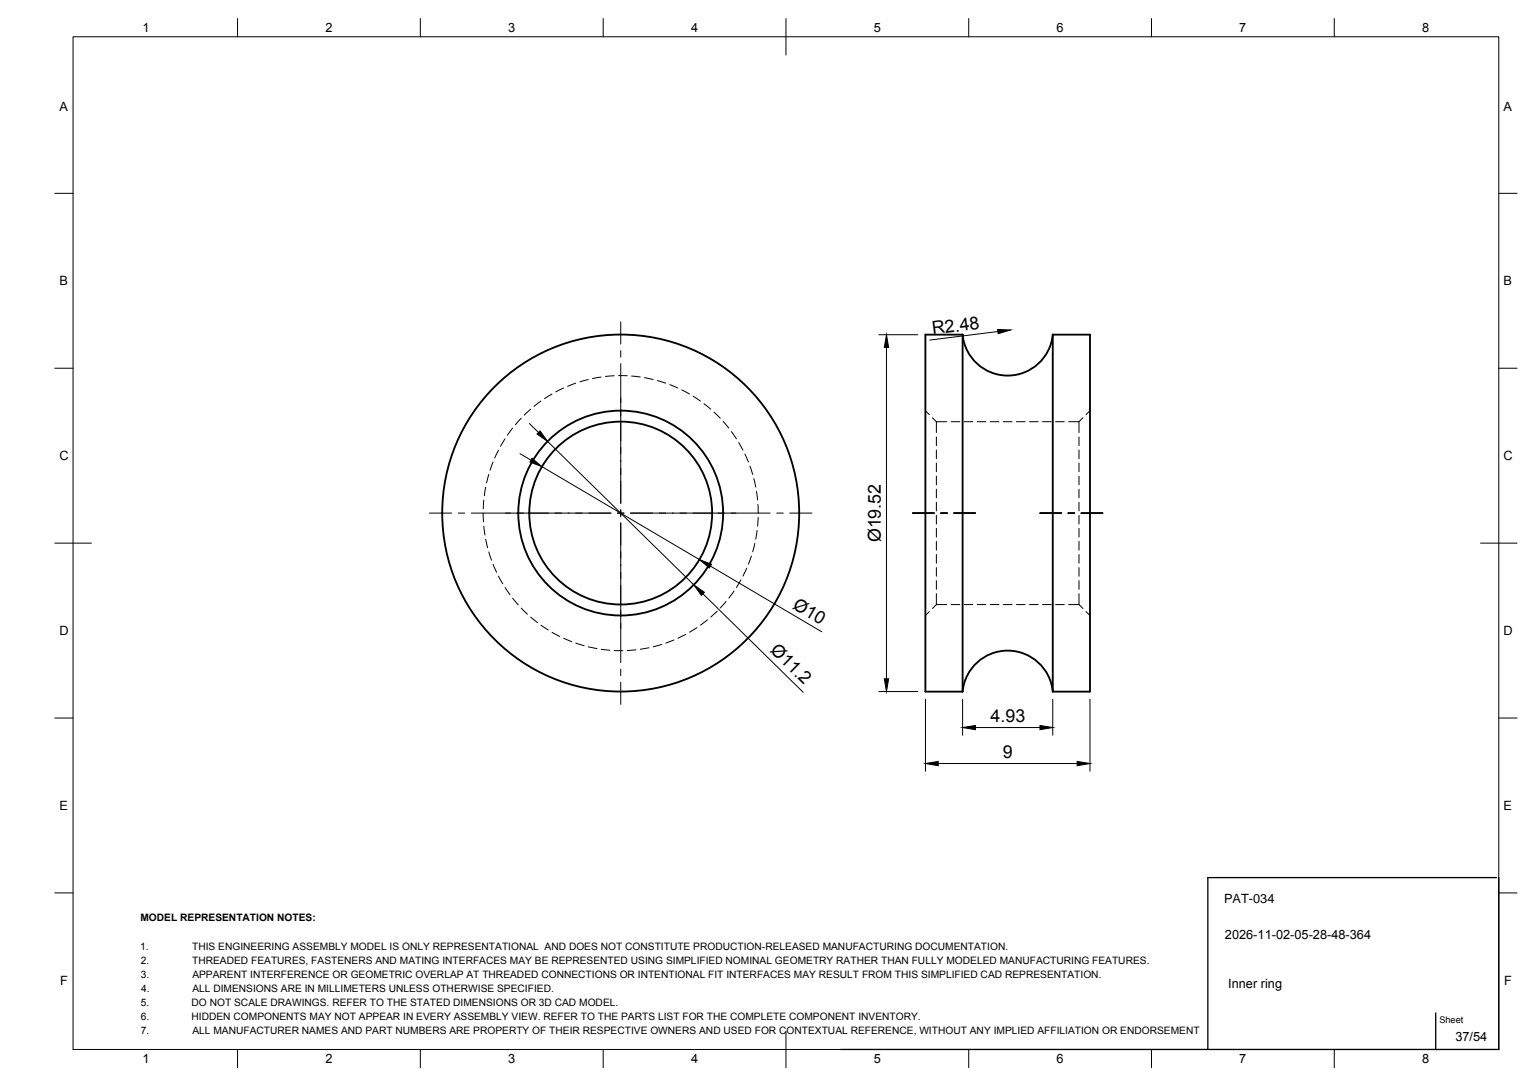
ISO-10303-21;
HEADER;
/* Generated by software containing ST-Developer
 * from STEP Tools, Inc. (www.steptools.com) 
 */

FILE_DESCRIPTION(
/* description */ ('Fatigue rig crank-slider'),
/* implementation_level */ '2;1');

FILE_NAME(
/* name */ 'Inner ring.step',
/* time_stamp */ '2026-10-28T03:24:50-07:00',
/* author */ (''),
/* organization */ (''),
/* preprocessor_version */ 'ST-DEVELOPER v20.2',
/* originating_system */ 'Autodesk Translation Framework v15.17.0.0',
/* authorisation */ '');

FILE_SCHEMA (('AUTOMOTIVE_DESIGN { 1 0 10303 214 3 1 1 }'));
ENDSEC;

DATA;
#10=MECHANICAL_DESIGN_GEOMETRIC_PRESENTATION_REPRESENTATION('',(#620),#16911);
#11=TOROIDAL_SURFACE('',#10108,1.,0.247676);
#22=CONICAL_SURFACE('',#10119,0.53,0.785398163397448);
#23=CONICAL_SURFACE('',#10126,0.53,0.785398163397448);
#519=SHAPE_REPRESENTATION_RELATIONSHIP('SRR','None',#17162,#569);
#569=ADVANCED_BREP_SHAPE_REPRESENTATION('',(#677),#16891);
#620=STYLED_ITEM('',(#17487),#677);
#677=MANIFOLD_SOLID_BREP('Body1',#8913);
#854=FACE_BOUND('',#2224,.T.);
#855=FACE_BOUND('',#2227,.T.);
#1094=PLANE('',#10121);
#1095=PLANE('',#10124);
#1542=FACE_OUTER_BOUND('',#2219,.T.);
#1543=FACE_OUTER_BOUND('',#2220,.T.);
#1544=FACE_OUTER_BOUND('',#2221,.T.);
#1545=FACE_OUTER_BOUND('',#2222,.T.);
#1546=FACE_OUTER_BOUND('',#2223,.T.);
#1547=FACE_OUTER_BOUND('',#2225,.T.);
#1548=FACE_OUTER_BOUND('',#2226,.T.);
#1549=FACE_OUTER_BOUND('',#2228,.T.);
#2219=EDGE_LOOP('',(#7340,#7341,#7342,#7343,#7344,#7345));
#2220=EDGE_LOOP('',(#7346,#7347,#7348,#7349,#7350));
#2221=EDGE_LOOP('',(#7351,#7352,#7353,#7354));
#2222=EDGE_LOOP('',(#7355,#7356,#7357,#7358));
#2223=EDGE_LOOP('',(#7359));
#2224=EDGE_LOOP('',(#7360));
#2225=EDGE_LOOP('',(#7361,#7362,#7363,#7364,#7365));
#2226=EDGE_LOOP('',(#7366));
#2227=EDGE_LOOP('',(#7367));
#2228=EDGE_LOOP('',(#7368,#7369,#7370,#7371));
#2847=LINE('',#15442,#3493);
#2848=LINE('',#15448,#3494);
#2849=LINE('',#15452,#3495);
#2850=LINE('',#15458,#3496);
#2851=LINE('',#15463,#3497);
#3493=VECTOR('',#12197,0.976185);
#3494=VECTOR('',#12204,0.5);
#3495=VECTOR('',#12209,0.53);
#3496=VECTOR('',#12218,0.976185);
#3497=VECTOR('',#12225,0.53);
#4001=CIRCLE('',#10109,0.976185);
#4002=CIRCLE('',#10110,0.976185);
#4003=CIRCLE('',#10111,0.247676);
#4004=CIRCLE('',#10112,0.976185);
#4005=CIRCLE('',#10113,0.976185);
#4006=CIRCLE('',#10115,0.976185);
#4007=CIRCLE('',#10117,0.5);
#4008=CIRCLE('',#10118,0.5);
#4009=CIRCLE('',#10120,0.56);
#4010=CIRCLE('',#10123,0.976185);
#4011=CIRCLE('',#10125,0.56);
#4605=VERTEX_POINT('',#15431);
#4606=VERTEX_POINT('',#15432);
#4607=VERTEX_POINT('',#15435);
#4608=VERTEX_POINT('',#15437);
#4609=VERTEX_POINT('',#15441);
#4610=VERTEX_POINT('',#15445);
#4611=VERTEX_POINT('',#15447);
#4612=VERTEX_POINT('',#15451);
#4613=VERTEX_POINT('',#15456);
#4614=VERTEX_POINT('',#15460);
#5568=EDGE_CURVE('',#4605,#4606,#4001,.T.);
#5569=EDGE_CURVE('',#4606,#4605,#4002,.T.);
#5570=EDGE_CURVE('',#4606,#4607,#4003,.T.);
#5571=EDGE_CURVE('',#4608,#4607,#4004,.T.);
#5572=EDGE_CURVE('',#4607,#4608,#4005,.T.);
#5573=EDGE_CURVE('',#4608,#4609,#2847,.T.);
#5574=EDGE_CURVE('',#4609,#4609,#4006,.T.);
#5575=EDGE_CURVE('',#4610,#4610,#4007,.T.);
#5576=EDGE_CURVE('',#4610,#4611,#2848,.T.);
#5577=EDGE_CURVE('',#4611,#4611,#4008,.T.);
#5578=EDGE_CURVE('',#4611,#4612,#2849,.T.);
#5579=EDGE_CURVE('',#4612,#4612,#4009,.T.);
#5580=EDGE_CURVE('',#4613,#4613,#4010,.T.);
#5581=EDGE_CURVE('',#4613,#4605,#2850,.T.);
#5582=EDGE_CURVE('',#4614,#4614,#4011,.T.);
#5583=EDGE_CURVE('',#4614,#4610,#2851,.T.);
#7340=ORIENTED_EDGE('',*,*,#5568,.F.);
#7341=ORIENTED_EDGE('',*,*,#5569,.F.);
#7342=ORIENTED_EDGE('',*,*,#5570,.T.);
#7343=ORIENTED_EDGE('',*,*,#5571,.F.);
#7344=ORIENTED_EDGE('',*,*,#5572,.F.);
#7345=ORIENTED_EDGE('',*,*,#5570,.F.);
#7346=ORIENTED_EDGE('',*,*,#5571,.T.);
#7347=ORIENTED_EDGE('',*,*,#5572,.T.);
#7348=ORIENTED_EDGE('',*,*,#5573,.T.);
#7349=ORIENTED_EDGE('',*,*,#5574,.T.);
#7350=ORIENTED_EDGE('',*,*,#5573,.F.);
#7351=ORIENTED_EDGE('',*,*,#5575,.T.);
#7352=ORIENTED_EDGE('',*,*,#5576,.T.);
#7353=ORIENTED_EDGE('',*,*,#5577,.F.);
#7354=ORIENTED_EDGE('',*,*,#5576,.F.);
#7355=ORIENTED_EDGE('',*,*,#5577,.T.);
#7356=ORIENTED_EDGE('',*,*,#5578,.T.);
#7357=ORIENTED_EDGE('',*,*,#5579,.F.);
#7358=ORIENTED_EDGE('',*,*,#5578,.F.);
#7359=ORIENTED_EDGE('',*,*,#5574,.F.);
#7360=ORIENTED_EDGE('',*,*,#5579,.T.);
#7361=ORIENTED_EDGE('',*,*,#5580,.F.);
#7362=ORIENTED_EDGE('',*,*,#5581,.T.);
#7363=ORIENTED_EDGE('',*,*,#5568,.T.);
#7364=ORIENTED_EDGE('',*,*,#5569,.T.);
#7365=ORIENTED_EDGE('',*,*,#5581,.F.);
#7366=ORIENTED_EDGE('',*,*,#5580,.T.);
#7367=ORIENTED_EDGE('',*,*,#5582,.F.);
#7368=ORIENTED_EDGE('',*,*,#5582,.T.);
#7369=ORIENTED_EDGE('',*,*,#5583,.T.);
#7370=ORIENTED_EDGE('',*,*,#5575,.F.);
#7371=ORIENTED_EDGE('',*,*,#5583,.F.);
#8313=CYLINDRICAL_SURFACE('',#10114,0.976185);
#8314=CYLINDRICAL_SURFACE('',#10116,0.5);
#8315=CYLINDRICAL_SURFACE('',#10122,0.976185);
#8680=ADVANCED_FACE('',(#1542),#11,.F.);
#8681=ADVANCED_FACE('',(#1543),#8313,.T.);
#8682=ADVANCED_FACE('',(#1544),#8314,.F.);
#8683=ADVANCED_FACE('',(#1545),#22,.F.);
#8684=ADVANCED_FACE('',(#1546,#854),#1094,.T.);
#8685=ADVANCED_FACE('',(#1547),#8315,.T.);
#8686=ADVANCED_FACE('',(#1548,#855),#1095,.T.);
#8687=ADVANCED_FACE('',(#1549),#23,.F.);
#8913=CLOSED_SHELL('',(#8680,#8681,#8682,#8683,#8684,#8685,#8686,#8687));
#10107=AXIS2_PLACEMENT_3D('',#15429,#12181,#12182);
#10108=AXIS2_PLACEMENT_3D('',#15430,#12183,#12184);
#10109=AXIS2_PLACEMENT_3D('',#15433,#12185,#12186);
#10110=AXIS2_PLACEMENT_3D('',#15434,#12187,#12188);
#10111=AXIS2_PLACEMENT_3D('',#15436,#12189,#12190);
#10112=AXIS2_PLACEMENT_3D('',#15438,#12191,#12192);
#10113=AXIS2_PLACEMENT_3D('',#15439,#12193,#12194);
#10114=AXIS2_PLACEMENT_3D('',#15440,#12195,#12196);
#10115=AXIS2_PLACEMENT_3D('',#15443,#12198,#12199);
#10116=AXIS2_PLACEMENT_3D('',#15444,#12200,#12201);
#10117=AXIS2_PLACEMENT_3D('',#15446,#12202,#12203);
#10118=AXIS2_PLACEMENT_3D('',#15449,#12205,#12206);
#10119=AXIS2_PLACEMENT_3D('',#15450,#12207,#12208);
#10120=AXIS2_PLACEMENT_3D('',#15453,#12210,#12211);
#10121=AXIS2_PLACEMENT_3D('',#15454,#12212,#12213);
#10122=AXIS2_PLACEMENT_3D('',#15455,#12214,#12215);
#10123=AXIS2_PLACEMENT_3D('',#15457,#12216,#12217);
#10124=AXIS2_PLACEMENT_3D('',#15459,#12219,#12220);
#10125=AXIS2_PLACEMENT_3D('',#15461,#12221,#12222);
#10126=AXIS2_PLACEMENT_3D('',#15462,#12223,#12224);
#12181=DIRECTION('axis',(0.,0.,1.));
#12182=DIRECTION('refdir',(1.,0.,0.));
#12183=DIRECTION('center_axis',(0.,-1.,0.));
#12184=DIRECTION('ref_axis',(0.,0.,-1.));
#12185=DIRECTION('center_axis',(0.,-1.,0.));
#12186=DIRECTION('ref_axis',(1.,0.,0.));
#12187=DIRECTION('center_axis',(0.,-1.,0.));
#12188=DIRECTION('ref_axis',(1.,0.,0.));
#12189=DIRECTION('center_axis',(1.,0.,1.22464679914735E-16));
#12190=DIRECTION('ref_axis',(-1.22464679914735E-16,0.,1.));
#12191=DIRECTION('center_axis',(0.,1.,0.));
#12192=DIRECTION('ref_axis',(1.,0.,0.));
#12193=DIRECTION('center_axis',(0.,1.,0.));
#12194=DIRECTION('ref_axis',(1.,0.,0.));
#12195=DIRECTION('center_axis',(0.,-1.,0.));
#12196=DIRECTION('ref_axis',(1.,0.,0.));
#12197=DIRECTION('',(0.,1.,0.));
#12198=DIRECTION('center_axis',(0.,-1.,0.));
#12199=DIRECTION('ref_axis',(1.,0.,0.));
#12200=DIRECTION('center_axis',(0.,-1.,0.));
#12201=DIRECTION('ref_axis',(1.,0.,0.));
#12202=DIRECTION('center_axis',(0.,-1.,0.));
#12203=DIRECTION('ref_axis',(1.,0.,0.));
#12204=DIRECTION('',(0.,1.,0.));
#12205=DIRECTION('center_axis',(0.,-1.,0.));
#12206=DIRECTION('ref_axis',(1.,0.,0.));
#12207=DIRECTION('center_axis',(0.,1.,0.));
#12208=DIRECTION('ref_axis',(1.,0.,0.));
#12209=DIRECTION('',(-0.707106781186547,0.707106781186548,-8.65956056235493E-17));
#12210=DIRECTION('center_axis',(0.,-1.,0.));
#12211=DIRECTION('ref_axis',(1.,0.,0.));
#12212=DIRECTION('center_axis',(0.,1.,0.));
#12213=DIRECTION('ref_axis',(0.,0.,1.));
#12214=DIRECTION('center_axis',(0.,-1.,0.));
#12215=DIRECTION('ref_axis',(1.,0.,0.));
#12216=DIRECTION('center_axis',(0.,-1.,0.));
#12217=DIRECTION('ref_axis',(1.,0.,0.));
#12218=DIRECTION('',(0.,1.,0.));
#12219=DIRECTION('center_axis',(0.,-1.,0.));
#12220=DIRECTION('ref_axis',(0.,0.,-1.));
#12221=DIRECTION('center_axis',(0.,-1.,0.));
#12222=DIRECTION('ref_axis',(1.,0.,0.));
#12223=DIRECTION('center_axis',(0.,-1.,0.));
#12224=DIRECTION('ref_axis',(1.,0.,0.));
#12225=DIRECTION('',(0.707106781186547,0.707106781186548,8.65956056235493E-17));
#15429=CARTESIAN_POINT('',(0.,0.,0.));
#15430=CARTESIAN_POINT('Origin',(0.,0.,0.));
#15431=CARTESIAN_POINT('',(-0.976185,-0.246528389340863,-1.19548183562566E-16));
#15432=CARTESIAN_POINT('',(-1.19548183562566E-16,-0.246528389340863,0.976185));
#15433=CARTESIAN_POINT('Origin',(0.,-0.246528389340863,0.));
#15434=CARTESIAN_POINT('Origin',(0.,-0.246528389340863,0.));
#15435=CARTESIAN_POINT('',(-1.19548183562566E-16,0.246528389340863,0.976185));
#15436=CARTESIAN_POINT('Origin',(-1.22464679914735E-16,0.,1.));
#15437=CARTESIAN_POINT('',(-0.976185,0.246528389340863,1.19548183562566E-16));
#15438=CARTESIAN_POINT('Origin',(0.,0.246528389340863,0.));
#15439=CARTESIAN_POINT('Origin',(0.,0.246528389340863,0.));
#15440=CARTESIAN_POINT('Origin',(0.,0.,0.));
#15441=CARTESIAN_POINT('',(-0.976185,0.45,-1.19548183562566E-16));
#15442=CARTESIAN_POINT('',(-0.976185,0.,-1.19548183562566E-16));
#15443=CARTESIAN_POINT('Origin',(0.,0.45,0.));
#15444=CARTESIAN_POINT('Origin',(0.,0.,0.));
#15445=CARTESIAN_POINT('',(-0.5,-0.39,-6.12323399573677E-17));
#15446=CARTESIAN_POINT('Origin',(0.,-0.39,0.));
#15447=CARTESIAN_POINT('',(-0.5,0.39,-6.12323399573677E-17));
#15448=CARTESIAN_POINT('',(-0.5,0.,-6.12323399573677E-17));
#15449=CARTESIAN_POINT('Origin',(0.,0.39,0.));
#15450=CARTESIAN_POINT('Origin',(0.,0.42,0.));
#15451=CARTESIAN_POINT('',(-0.56,0.45,-6.85802207522518E-17));
#15452=CARTESIAN_POINT('',(-0.53,0.42,-6.49062803548097E-17));
#15453=CARTESIAN_POINT('Origin',(0.,0.45,0.));
#15454=CARTESIAN_POINT('Origin',(0.976185,0.45,0.));
#15455=CARTESIAN_POINT('Origin',(0.,0.,0.));
#15456=CARTESIAN_POINT('',(-0.976185,-0.45,-1.19548183562566E-16));
#15457=CARTESIAN_POINT('Origin',(0.,-0.45,0.));
#15458=CARTESIAN_POINT('',(-0.976185,0.,-1.19548183562566E-16));
#15459=CARTESIAN_POINT('Origin',(0.56,-0.45,0.));
#15460=CARTESIAN_POINT('',(-0.56,-0.45,-6.85802207522518E-17));
#15461=CARTESIAN_POINT('Origin',(0.,-0.45,0.));
#15462=CARTESIAN_POINT('Origin',(0.,-0.42,0.));
#15463=CARTESIAN_POINT('',(-0.53,-0.42,-6.49062803548097E-17));
#16832=UNCERTAINTY_MEASURE_WITH_UNIT(LENGTH_MEASURE(0.001),#16912,
'DISTANCE_ACCURACY_VALUE',
'Maximum model space distance between geometric entities at asserted c
onnectivities');
#16852=UNCERTAINTY_MEASURE_WITH_UNIT(LENGTH_MEASURE(0.001),#16912,
'DISTANCE_ACCURACY_VALUE',
'Maximum model space distance between geometric entities at asserted c
onnectivities');
#16891=(
GEOMETRIC_REPRESENTATION_CONTEXT(3)
GLOBAL_UNCERTAINTY_ASSIGNED_CONTEXT((#16832))
GLOBAL_UNIT_ASSIGNED_CONTEXT((#16912,#16914,#16915))
REPRESENTATION_CONTEXT('','3D')
);
#16911=(
GEOMETRIC_REPRESENTATION_CONTEXT(3)
GLOBAL_UNCERTAINTY_ASSIGNED_CONTEXT((#16852))
GLOBAL_UNIT_ASSIGNED_CONTEXT((#16912,#16914,#16915))
REPRESENTATION_CONTEXT('','3D')
);
#16912=(
LENGTH_UNIT()
NAMED_UNIT(*)
SI_UNIT(.CENTI.,.METRE.)
);
#16914=(
NAMED_UNIT(*)
PLANE_ANGLE_UNIT()
SI_UNIT($,.RADIAN.)
);
#16915=(
NAMED_UNIT(*)
SI_UNIT($,.STERADIAN.)
SOLID_ANGLE_UNIT()
);
#16954=SHAPE_DEFINITION_REPRESENTATION(#17014,#17162);
#17014=PRODUCT_DEFINITION_SHAPE('',$,#17221);
#17162=SHAPE_REPRESENTATION('',(#10107),#16891);
#17182=PRODUCT_DEFINITION_CONTEXT('part definition',#17358,'design');
#17221=PRODUCT_DEFINITION('Inner ring','Inner ring',#17279,#17182);
#17279=PRODUCT_DEFINITION_FORMATION('',$,#17398);
#17358=APPLICATION_CONTEXT(
'Core Data for Automotive Mechanical Design Process');
#17359=PRODUCT_CONTEXT('part definition',#17358,'mechanical');
#17398=PRODUCT('Inner ring','Inner ring','Inner ring',(#17359));
#17481=COLOUR_RGB('Grey',0.48,0.52,0.57);
#17482=FILL_AREA_STYLE_COLOUR('',#17481);
#17483=FILL_AREA_STYLE('',(#17482));
#17484=SURFACE_STYLE_FILL_AREA(#17483);
#17485=SURFACE_SIDE_STYLE('',(#17484));
#17486=SURFACE_STYLE_USAGE(.BOTH.,#17485);
#17487=PRESENTATION_STYLE_ASSIGNMENT((#17486));
ENDSEC;
END-ISO-10303-21;
